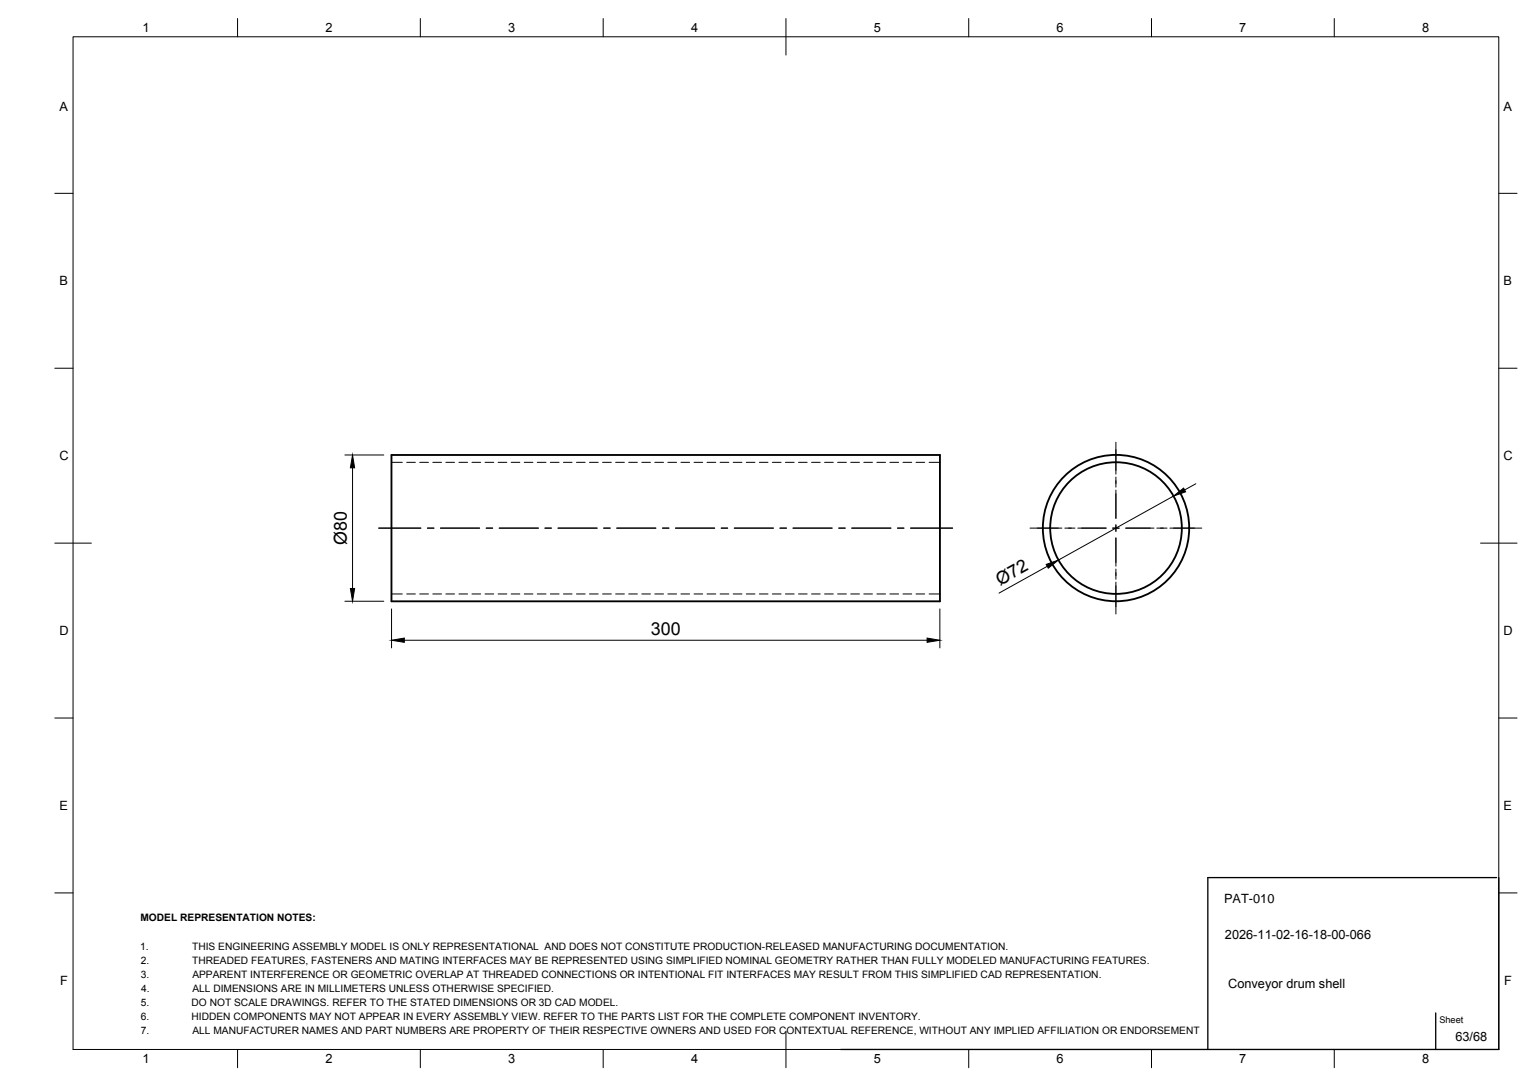
ISO-10303-21;
HEADER;
/* Generated by software containing ST-Developer
 * from STEP Tools, Inc. (www.steptools.com) 
 */

FILE_DESCRIPTION(
/* description */ ('Belt conveyor head drive unit'),
/* implementation_level */ '2;1');

FILE_NAME(
/* name */ 'Conveyor drum shell.step',
/* time_stamp */ '2026-10-28T03:26:19-07:00',
/* author */ (''),
/* organization */ (''),
/* preprocessor_version */ 'ST-DEVELOPER v20.2',
/* originating_system */ 'Autodesk Translation Framework v15.17.0.0',
/* authorisation */ '');

FILE_SCHEMA (('AUTOMOTIVE_DESIGN { 1 0 10303 214 3 1 1 }'));
ENDSEC;

DATA;
#10=MECHANICAL_DESIGN_GEOMETRIC_PRESENTATION_REPRESENTATION('',(#924),#27069);
#770=SHAPE_REPRESENTATION_RELATIONSHIP('SRR','None',#27419,#839);
#839=ADVANCED_BREP_SHAPE_REPRESENTATION('',(#1005),#27061);
#924=STYLED_ITEM('',(#27811),#1005);
#1005=MANIFOLD_SOLID_BREP('Body1',#13793);
#1250=FACE_BOUND('',#3326,.T.);
#1251=FACE_BOUND('',#3328,.T.);
#1594=PLANE('',#15966);
#1595=PLANE('',#15967);
#2285=FACE_OUTER_BOUND('',#3323,.T.);
#2286=FACE_OUTER_BOUND('',#3324,.T.);
#2287=FACE_OUTER_BOUND('',#3325,.T.);
#2288=FACE_OUTER_BOUND('',#3327,.T.);
#3323=EDGE_LOOP('',(#11758,#11759,#11760,#11761));
#3324=EDGE_LOOP('',(#11762,#11763,#11764,#11765));
#3325=EDGE_LOOP('',(#11766));
#3326=EDGE_LOOP('',(#11767));
#3327=EDGE_LOOP('',(#11768));
#3328=EDGE_LOOP('',(#11769));
#4139=LINE('',#25607,#4931);
#4140=LINE('',#25613,#4932);
#4931=VECTOR('',#19875,3.6);
#4932=VECTOR('',#19882,4.);
#5747=CIRCLE('',#15961,3.6);
#5748=CIRCLE('',#15962,3.6);
#5749=CIRCLE('',#15964,4.);
#5750=CIRCLE('',#15965,4.);
#6911=VERTEX_POINT('',#25604);
#6912=VERTEX_POINT('',#25606);
#6913=VERTEX_POINT('',#25610);
#6914=VERTEX_POINT('',#25612);
#8571=EDGE_CURVE('',#6911,#6911,#5747,.T.);
#8572=EDGE_CURVE('',#6911,#6912,#4139,.T.);
#8573=EDGE_CURVE('',#6912,#6912,#5748,.T.);
#8574=EDGE_CURVE('',#6913,#6913,#5749,.T.);
#8575=EDGE_CURVE('',#6913,#6914,#4140,.T.);
#8576=EDGE_CURVE('',#6914,#6914,#5750,.T.);
#11758=ORIENTED_EDGE('',*,*,#8571,.F.);
#11759=ORIENTED_EDGE('',*,*,#8572,.T.);
#11760=ORIENTED_EDGE('',*,*,#8573,.T.);
#11761=ORIENTED_EDGE('',*,*,#8572,.F.);
#11762=ORIENTED_EDGE('',*,*,#8574,.F.);
#11763=ORIENTED_EDGE('',*,*,#8575,.T.);
#11764=ORIENTED_EDGE('',*,*,#8576,.T.);
#11765=ORIENTED_EDGE('',*,*,#8575,.F.);
#11766=ORIENTED_EDGE('',*,*,#8574,.T.);
#11767=ORIENTED_EDGE('',*,*,#8571,.T.);
#11768=ORIENTED_EDGE('',*,*,#8576,.F.);
#11769=ORIENTED_EDGE('',*,*,#8573,.F.);
#12809=CYLINDRICAL_SURFACE('',#15960,3.6);
#12810=CYLINDRICAL_SURFACE('',#15963,4.);
#13564=ADVANCED_FACE('',(#2285),#12809,.F.);
#13565=ADVANCED_FACE('',(#2286),#12810,.T.);
#13566=ADVANCED_FACE('',(#2287,#1250),#1594,.T.);
#13567=ADVANCED_FACE('',(#2288,#1251),#1595,.F.);
#13793=CLOSED_SHELL('',(#13564,#13565,#13566,#13567));
#15959=AXIS2_PLACEMENT_3D('',#25602,#19869,#19870);
#15960=AXIS2_PLACEMENT_3D('',#25603,#19871,#19872);
#15961=AXIS2_PLACEMENT_3D('',#25605,#19873,#19874);
#15962=AXIS2_PLACEMENT_3D('',#25608,#19876,#19877);
#15963=AXIS2_PLACEMENT_3D('',#25609,#19878,#19879);
#15964=AXIS2_PLACEMENT_3D('',#25611,#19880,#19881);
#15965=AXIS2_PLACEMENT_3D('',#25614,#19883,#19884);
#15966=AXIS2_PLACEMENT_3D('',#25615,#19885,#19886);
#15967=AXIS2_PLACEMENT_3D('',#25616,#19887,#19888);
#19869=DIRECTION('axis',(0.,0.,1.));
#19870=DIRECTION('refdir',(1.,0.,0.));
#19871=DIRECTION('center_axis',(0.,1.,0.));
#19872=DIRECTION('ref_axis',(1.,0.,0.));
#19873=DIRECTION('center_axis',(0.,-1.,0.));
#19874=DIRECTION('ref_axis',(1.,0.,0.));
#19875=DIRECTION('',(0.,-1.,0.));
#19876=DIRECTION('center_axis',(0.,-1.,0.));
#19877=DIRECTION('ref_axis',(1.,0.,0.));
#19878=DIRECTION('center_axis',(0.,1.,0.));
#19879=DIRECTION('ref_axis',(1.,0.,0.));
#19880=DIRECTION('center_axis',(0.,1.,0.));
#19881=DIRECTION('ref_axis',(1.,0.,0.));
#19882=DIRECTION('',(0.,-1.,0.));
#19883=DIRECTION('center_axis',(0.,1.,0.));
#19884=DIRECTION('ref_axis',(1.,0.,0.));
#19885=DIRECTION('center_axis',(0.,1.,0.));
#19886=DIRECTION('ref_axis',(1.,0.,0.));
#19887=DIRECTION('center_axis',(0.,1.,0.));
#19888=DIRECTION('ref_axis',(1.,0.,0.));
#25602=CARTESIAN_POINT('',(0.,0.,0.));
#25603=CARTESIAN_POINT('Origin',(6.97091003018116,7.,7.));
#25604=CARTESIAN_POINT('',(3.37091003018116,37.,7.));
#25605=CARTESIAN_POINT('Origin',(6.97091003018116,37.,7.));
#25606=CARTESIAN_POINT('',(3.37091003018116,7.,7.));
#25607=CARTESIAN_POINT('',(3.37091003018116,7.,7.));
#25608=CARTESIAN_POINT('Origin',(6.97091003018116,7.,7.));
#25609=CARTESIAN_POINT('Origin',(6.97091003018116,7.,7.));
#25610=CARTESIAN_POINT('',(2.97091003018116,37.,7.));
#25611=CARTESIAN_POINT('Origin',(6.97091003018116,37.,7.));
#25612=CARTESIAN_POINT('',(2.97091003018116,7.,7.));
#25613=CARTESIAN_POINT('',(2.97091003018116,7.,7.));
#25614=CARTESIAN_POINT('Origin',(6.97091003018116,7.,7.));
#25615=CARTESIAN_POINT('Origin',(6.97091003018116,37.,7.));
#25616=CARTESIAN_POINT('Origin',(6.97091003018116,7.,7.));
#26984=UNCERTAINTY_MEASURE_WITH_UNIT(LENGTH_MEASURE(0.001),#27070,
'DISTANCE_ACCURACY_VALUE',
'Maximum model space distance between geometric entities at asserted c
onnectivities');
#26992=UNCERTAINTY_MEASURE_WITH_UNIT(LENGTH_MEASURE(0.001),#27070,
'DISTANCE_ACCURACY_VALUE',
'Maximum model space distance between geometric entities at asserted c
onnectivities');
#27061=(
GEOMETRIC_REPRESENTATION_CONTEXT(3)
GLOBAL_UNCERTAINTY_ASSIGNED_CONTEXT((#26984))
GLOBAL_UNIT_ASSIGNED_CONTEXT((#27070,#27072,#27073))
REPRESENTATION_CONTEXT('','3D')
);
#27069=(
GEOMETRIC_REPRESENTATION_CONTEXT(3)
GLOBAL_UNCERTAINTY_ASSIGNED_CONTEXT((#26992))
GLOBAL_UNIT_ASSIGNED_CONTEXT((#27070,#27072,#27073))
REPRESENTATION_CONTEXT('','3D')
);
#27070=(
LENGTH_UNIT()
NAMED_UNIT(*)
SI_UNIT(.CENTI.,.METRE.)
);
#27072=(
NAMED_UNIT(*)
PLANE_ANGLE_UNIT()
SI_UNIT($,.RADIAN.)
);
#27073=(
NAMED_UNIT(*)
SI_UNIT($,.STERADIAN.)
SOLID_ANGLE_UNIT()
);
#27142=SHAPE_DEFINITION_REPRESENTATION(#27230,#27419);
#27230=PRODUCT_DEFINITION_SHAPE('',$,#27496);
#27419=SHAPE_REPRESENTATION('',(#15959),#27061);
#27427=PRODUCT_DEFINITION_CONTEXT('part definition',#27657,'design');
#27496=PRODUCT_DEFINITION('Conveyor drum shell','Conveyor drum shell',#27572,
#27427);
#27572=PRODUCT_DEFINITION_FORMATION('',$,#27727);
#27657=APPLICATION_CONTEXT(
'Core Data for Automotive Mechanical Design Process');
#27658=PRODUCT_CONTEXT('part definition',#27657,'mechanical');
#27727=PRODUCT('Conveyor drum shell','Conveyor drum shell',
'Conveyor drum shell',(#27658));
#27805=COLOUR_RGB('Off White',0.89,0.88,0.83);
#27806=FILL_AREA_STYLE_COLOUR('',#27805);
#27807=FILL_AREA_STYLE('',(#27806));
#27808=SURFACE_STYLE_FILL_AREA(#27807);
#27809=SURFACE_SIDE_STYLE('',(#27808));
#27810=SURFACE_STYLE_USAGE(.BOTH.,#27809);
#27811=PRESENTATION_STYLE_ASSIGNMENT((#27810));
ENDSEC;
END-ISO-10303-21;
